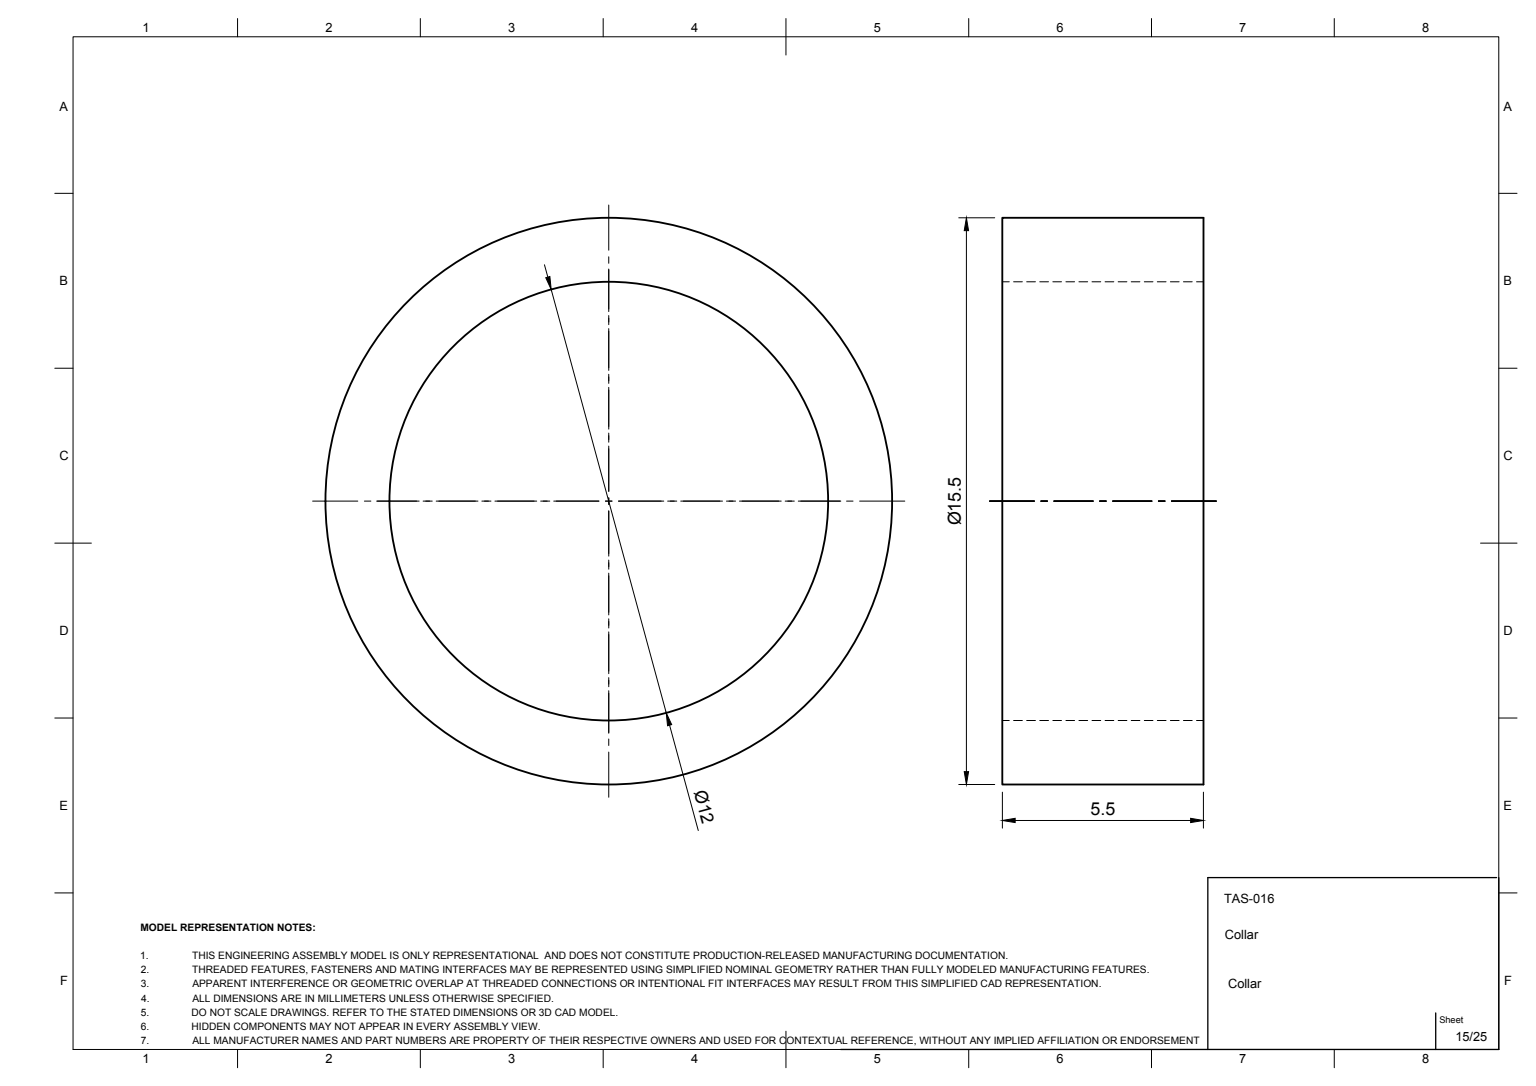
ISO-10303-21;
HEADER;
/* Generated by software containing ST-Developer
 * from STEP Tools, Inc. (www.steptools.com) 
 */

FILE_DESCRIPTION(
/* description */ ('STEP AP214'),
/* implementation_level */ '2;1');

FILE_NAME(
/* name */ 'Collar.step',
/* time_stamp */ '2026-11-15T14:55:55-08:00',
/* author */ (''),
/* organization */ (''),
/* preprocessor_version */ 'ST-DEVELOPER v20.2',
/* originating_system */ 'Autodesk Translation Framework v15.17.0.0',
/* authorisation */ '');

FILE_SCHEMA (('AUTOMOTIVE_DESIGN { 1 0 10303 214 3 1 1 }'));
ENDSEC;

DATA;
#10=MECHANICAL_DESIGN_GEOMETRIC_PRESENTATION_REPRESENTATION('',(#932),#57079);
#873=SHAPE_REPRESENTATION_RELATIONSHIP('SRR','None',#57258,#902);
#902=ADVANCED_BREP_SHAPE_REPRESENTATION('',(#969),#57050);
#932=STYLED_ITEM('',(#57444),#969);
#969=MANIFOLD_SOLID_BREP('Body1',#24532);
#1075=FACE_BOUND('',#3822,.T.);
#1076=FACE_BOUND('',#3824,.T.);
#1470=PLANE('',#25270);
#1471=PLANE('',#25271);
#2369=FACE_OUTER_BOUND('',#3819,.T.);
#2370=FACE_OUTER_BOUND('',#3820,.T.);
#2371=FACE_OUTER_BOUND('',#3821,.T.);
#2372=FACE_OUTER_BOUND('',#3823,.T.);
#3819=EDGE_LOOP('',(#16858,#16859,#16860,#16861));
#3820=EDGE_LOOP('',(#16862,#16863,#16864,#16865));
#3821=EDGE_LOOP('',(#16866));
#3822=EDGE_LOOP('',(#16867));
#3823=EDGE_LOOP('',(#16868));
#3824=EDGE_LOOP('',(#16869));
#5548=LINE('',#35862,#7515);
#5549=LINE('',#35868,#7516);
#7515=VECTOR('',#28540,7.75);
#7516=VECTOR('',#28547,6.);
#9344=CIRCLE('',#25265,7.75);
#9345=CIRCLE('',#25266,7.75);
#9346=CIRCLE('',#25268,6.);
#9347=CIRCLE('',#25269,6.);
#10585=VERTEX_POINT('',#35859);
#10586=VERTEX_POINT('',#35861);
#10587=VERTEX_POINT('',#35865);
#10588=VERTEX_POINT('',#35867);
#12974=EDGE_CURVE('',#10585,#10585,#9344,.T.);
#12975=EDGE_CURVE('',#10585,#10586,#5548,.T.);
#12976=EDGE_CURVE('',#10586,#10586,#9345,.T.);
#12977=EDGE_CURVE('',#10587,#10587,#9346,.T.);
#12978=EDGE_CURVE('',#10587,#10588,#5549,.T.);
#12979=EDGE_CURVE('',#10588,#10588,#9347,.T.);
#16858=ORIENTED_EDGE('',*,*,#12974,.F.);
#16859=ORIENTED_EDGE('',*,*,#12975,.T.);
#16860=ORIENTED_EDGE('',*,*,#12976,.T.);
#16861=ORIENTED_EDGE('',*,*,#12975,.F.);
#16862=ORIENTED_EDGE('',*,*,#12977,.F.);
#16863=ORIENTED_EDGE('',*,*,#12978,.T.);
#16864=ORIENTED_EDGE('',*,*,#12979,.T.);
#16865=ORIENTED_EDGE('',*,*,#12978,.F.);
#16866=ORIENTED_EDGE('',*,*,#12974,.T.);
#16867=ORIENTED_EDGE('',*,*,#12979,.F.);
#16868=ORIENTED_EDGE('',*,*,#12976,.F.);
#16869=ORIENTED_EDGE('',*,*,#12977,.T.);
#22799=CYLINDRICAL_SURFACE('',#25264,7.75);
#22800=CYLINDRICAL_SURFACE('',#25267,6.);
#23361=ADVANCED_FACE('',(#2369),#22799,.T.);
#23362=ADVANCED_FACE('',(#2370),#22800,.F.);
#23363=ADVANCED_FACE('',(#2371,#1075),#1470,.F.);
#23364=ADVANCED_FACE('',(#2372,#1076),#1471,.F.);
#24532=CLOSED_SHELL('',(#23361,#23362,#23363,#23364));
#25263=AXIS2_PLACEMENT_3D('',#35857,#28534,#28535);
#25264=AXIS2_PLACEMENT_3D('',#35858,#28536,#28537);
#25265=AXIS2_PLACEMENT_3D('',#35860,#28538,#28539);
#25266=AXIS2_PLACEMENT_3D('',#35863,#28541,#28542);
#25267=AXIS2_PLACEMENT_3D('',#35864,#28543,#28544);
#25268=AXIS2_PLACEMENT_3D('',#35866,#28545,#28546);
#25269=AXIS2_PLACEMENT_3D('',#35869,#28548,#28549);
#25270=AXIS2_PLACEMENT_3D('',#35870,#28550,#28551);
#25271=AXIS2_PLACEMENT_3D('',#35871,#28552,#28553);
#28534=DIRECTION('axis',(0.,0.,1.));
#28535=DIRECTION('refdir',(1.,0.,0.));
#28536=DIRECTION('center_axis',(-1.,0.,0.));
#28537=DIRECTION('ref_axis',(0.,0.,1.));
#28538=DIRECTION('center_axis',(-1.,0.,0.));
#28539=DIRECTION('ref_axis',(0.,0.,1.));
#28540=DIRECTION('',(1.,0.,0.));
#28541=DIRECTION('center_axis',(-1.,0.,0.));
#28542=DIRECTION('ref_axis',(0.,0.,1.));
#28543=DIRECTION('center_axis',(-1.,0.,0.));
#28544=DIRECTION('ref_axis',(0.,0.,1.));
#28545=DIRECTION('center_axis',(-1.,0.,0.));
#28546=DIRECTION('ref_axis',(0.,0.,1.));
#28547=DIRECTION('',(-1.,0.,0.));
#28548=DIRECTION('center_axis',(-1.,0.,0.));
#28549=DIRECTION('ref_axis',(0.,0.,1.));
#28550=DIRECTION('center_axis',(1.,0.,0.));
#28551=DIRECTION('ref_axis',(0.,0.,-1.));
#28552=DIRECTION('center_axis',(-1.,0.,0.));
#28553=DIRECTION('ref_axis',(0.,0.,1.));
#35857=CARTESIAN_POINT('',(0.,0.,0.));
#35858=CARTESIAN_POINT('Origin',(-0.25,0.,0.));
#35859=CARTESIAN_POINT('',(-3.81639164714898E-16,-9.49101269339199E-16,
-7.75));
#35860=CARTESIAN_POINT('Origin',(-3.79470760369927E-16,0.,0.));
#35861=CARTESIAN_POINT('',(5.5,-9.49101269339199E-16,-7.75));
#35862=CARTESIAN_POINT('',(-0.25,-9.49101269339199E-16,-7.75));
#35863=CARTESIAN_POINT('Origin',(5.5,0.,0.));
#35864=CARTESIAN_POINT('Origin',(-0.25,0.,0.));
#35865=CARTESIAN_POINT('',(5.5,-7.34788079488412E-16,-6.));
#35866=CARTESIAN_POINT('Origin',(5.5,0.,0.));
#35867=CARTESIAN_POINT('',(0.,-7.34788079488412E-16,-6.));
#35868=CARTESIAN_POINT('',(-0.25,-7.34788079488412E-16,-6.));
#35869=CARTESIAN_POINT('Origin',(0.,0.,0.));
#35870=CARTESIAN_POINT('Origin',(-1.83697019872103E-16,7.75,0.));
#35871=CARTESIAN_POINT('Origin',(5.5,6.,0.));
#57011=UNCERTAINTY_MEASURE_WITH_UNIT(LENGTH_MEASURE(0.01),#57080,
'DISTANCE_ACCURACY_VALUE',
'Maximum model space distance between geometric entities at asserted c
onnectivities');
#57040=UNCERTAINTY_MEASURE_WITH_UNIT(LENGTH_MEASURE(0.01),#57080,
'DISTANCE_ACCURACY_VALUE',
'Maximum model space distance between geometric entities at asserted c
onnectivities');
#57050=(
GEOMETRIC_REPRESENTATION_CONTEXT(3)
GLOBAL_UNCERTAINTY_ASSIGNED_CONTEXT((#57011))
GLOBAL_UNIT_ASSIGNED_CONTEXT((#57080,#57082,#57083))
REPRESENTATION_CONTEXT('','3D')
);
#57079=(
GEOMETRIC_REPRESENTATION_CONTEXT(3)
GLOBAL_UNCERTAINTY_ASSIGNED_CONTEXT((#57040))
GLOBAL_UNIT_ASSIGNED_CONTEXT((#57080,#57082,#57083))
REPRESENTATION_CONTEXT('','3D')
);
#57080=(
LENGTH_UNIT()
NAMED_UNIT(*)
SI_UNIT(.MILLI.,.METRE.)
);
#57082=(
NAMED_UNIT(*)
PLANE_ANGLE_UNIT()
SI_UNIT($,.RADIAN.)
);
#57083=(
NAMED_UNIT(*)
SI_UNIT($,.STERADIAN.)
SOLID_ANGLE_UNIT()
);
#57093=SHAPE_DEFINITION_REPRESENTATION(#57133,#57258);
#57133=PRODUCT_DEFINITION_SHAPE('',$,#57297);
#57258=SHAPE_REPRESENTATION('',(#25263),#57050);
#57287=PRODUCT_DEFINITION_CONTEXT('part definition',#57403,'design');
#57297=PRODUCT_DEFINITION('Collar','Collar',#57335,#57287);
#57335=PRODUCT_DEFINITION_FORMATION('',$,#57414);
#57403=APPLICATION_CONTEXT(
'Core Data for Automotive Mechanical Design Process');
#57404=PRODUCT_CONTEXT('part definition',#57403,'mechanical');
#57414=PRODUCT('Collar','Collar',$,(#57404));
#57444=PRESENTATION_STYLE_ASSIGNMENT((#57446));
#57446=SURFACE_STYLE_USAGE(.BOTH.,#57448);
#57448=SURFACE_SIDE_STYLE('',(#57450));
#57450=SURFACE_STYLE_FILL_AREA(#57452);
#57452=FILL_AREA_STYLE('Opaque(202,209,238)',(#57454));
#57454=FILL_AREA_STYLE_COLOUR('Opaque(202,209,238)',#57456);
#57456=COLOUR_RGB('Opaque(202,209,238)',0.792156862745098,0.819607843137255,
0.933333333333333);
ENDSEC;
END-ISO-10303-21;
